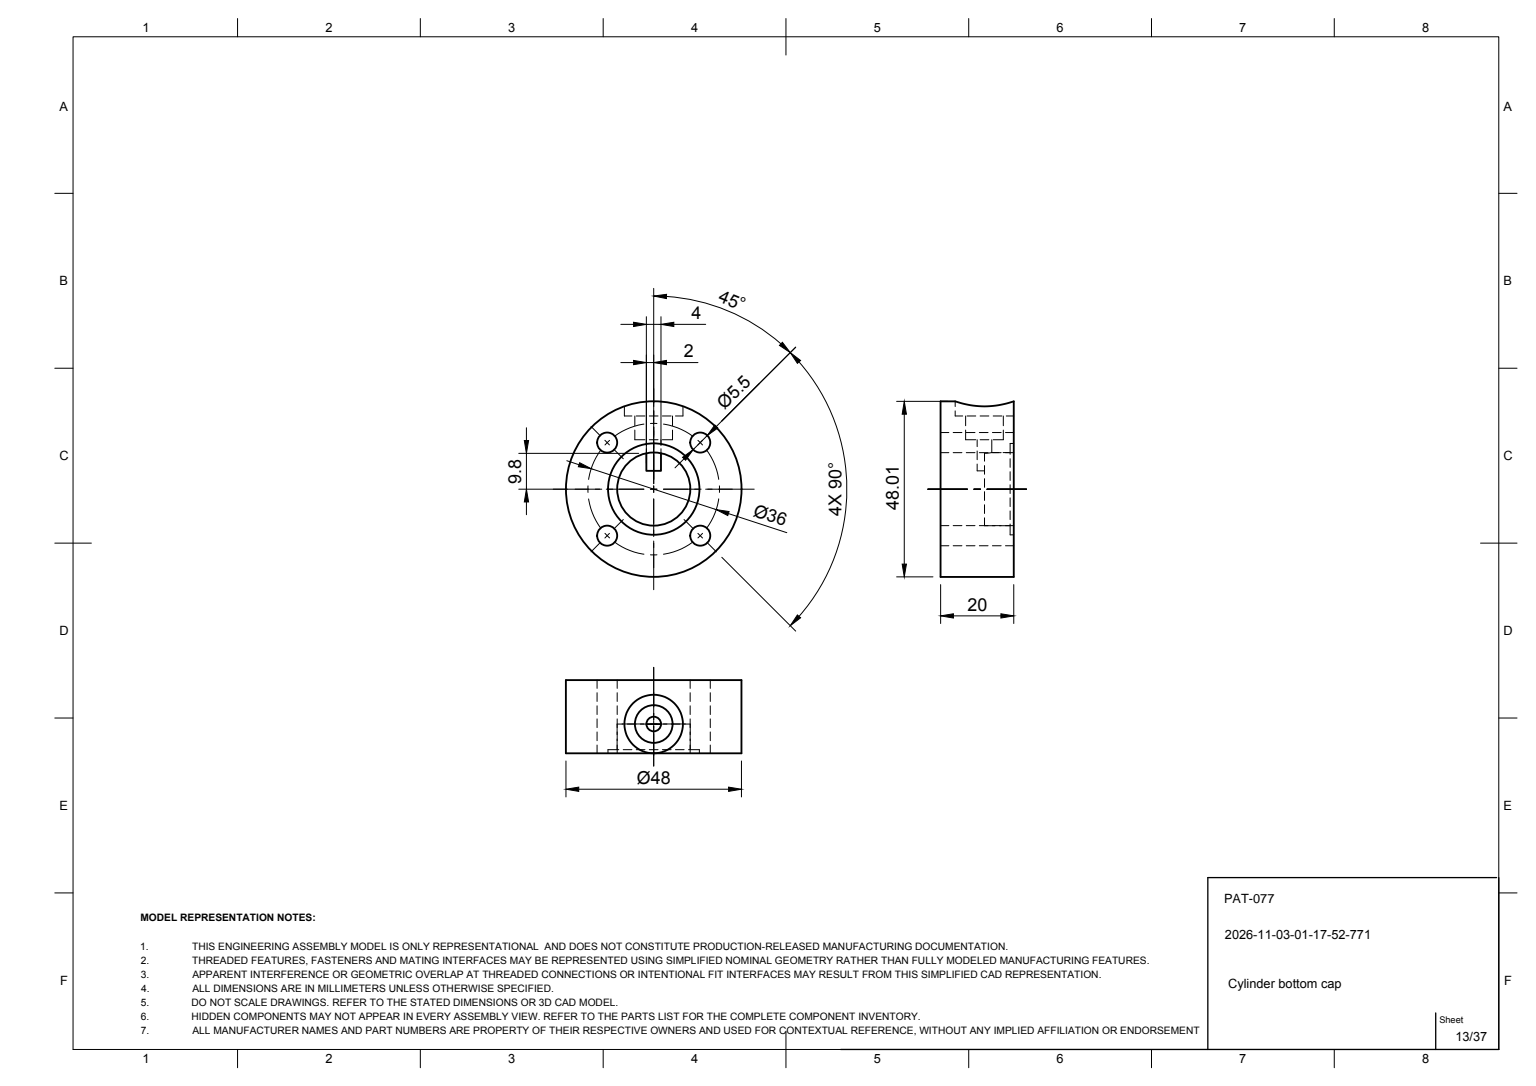
ISO-10303-21;
HEADER;
/* Generated by software containing ST-Developer
 * from STEP Tools, Inc. (www.steptools.com) 
 */

FILE_DESCRIPTION(
/* description */ ('Pallet stop with pneumatic fitting'),
/* implementation_level */ '2;1');

FILE_NAME(
/* name */ 'Cylinder bottom cap.step',
/* time_stamp */ '2026-10-27T10:51:41-07:00',
/* author */ (''),
/* organization */ (''),
/* preprocessor_version */ 'ST-DEVELOPER v20.2',
/* originating_system */ 'Autodesk Translation Framework v15.17.0.0',
/* authorisation */ '');

FILE_SCHEMA (('AUTOMOTIVE_DESIGN { 1 0 10303 214 3 1 1 }'));
ENDSEC;

DATA;
#10=MECHANICAL_DESIGN_GEOMETRIC_PRESENTATION_REPRESENTATION('',(#365),#10265);
#281=B_SPLINE_CURVE_WITH_KNOTS('',3,(#8964,#8965,#8966,#8967,#8968,#8969,
#8970,#8971,#8972,#8973,#8974,#8975,#8976,#8977,#8978,#8979,#8980,#8981,
#8982,#8983,#8984,#8985,#8986,#8987,#8988,#8989),.UNSPECIFIED.,.F.,.F.,
(4,2,2,2,2,2,2,2,2,2,2,2,4),(4.86208093968474,5.16603148466369,5.46998202964264,
5.77379160212428,6.07760117460592,6.38141074708757,6.68522031956921,6.98917086454816,
7.29312140952711,7.59707195450606,7.90102249948501,8.20483207196665,8.50864164444829),
 .UNSPECIFIED.);
#282=B_SPLINE_CURVE_WITH_KNOTS('',3,(#8999,#9000,#9001,#9002,#9003,#9004,
#9005,#9006,#9007,#9008,#9009,#9010,#9011,#9012,#9013,#9014,#9015,#9016),
 .UNSPECIFIED.,.F.,.F.,(4,2,2,2,2,2,2,2,4),(0.,0.0755590511780388,0.151118102356078,
0.226672919608918,0.302227736861757,0.377782554114597,0.453337371367437,
0.528896422545476,0.604455473723515),.UNSPECIFIED.);
#283=B_SPLINE_CURVE_WITH_KNOTS('',3,(#9033,#9034,#9035,#9036,#9037,#9038,
#9039,#9040,#9041,#9042),.UNSPECIFIED.,.F.,.F.,(4,2,2,2,4),(3.64656070476355,
3.9503702772452,4.25417984972684,4.55813039470579,4.86208093968474),
 .UNSPECIFIED.);
#301=SHAPE_REPRESENTATION_RELATIONSHIP('SRR','None',#10414,#333);
#333=ADVANCED_BREP_SHAPE_REPRESENTATION('',(#397),#10238);
#365=STYLED_ITEM('',(#10648),#397);
#397=MANIFOLD_SOLID_BREP('Body1',#5053);
#466=FACE_BOUND('',#1191,.T.);
#467=FACE_BOUND('',#1194,.T.);
#468=FACE_BOUND('',#1198,.T.);
#469=FACE_BOUND('',#1205,.T.);
#470=FACE_BOUND('',#1206,.T.);
#471=FACE_BOUND('',#1207,.T.);
#472=FACE_BOUND('',#1208,.T.);
#473=FACE_BOUND('',#1209,.T.);
#474=FACE_BOUND('',#1211,.T.);
#475=FACE_BOUND('',#1212,.T.);
#476=FACE_BOUND('',#1213,.T.);
#477=FACE_BOUND('',#1214,.T.);
#599=PLANE('',#5600);
#600=PLANE('',#5604);
#601=PLANE('',#5610);
#602=PLANE('',#5613);
#603=PLANE('',#5621);
#604=PLANE('',#5636);
#605=PLANE('',#5637);
#824=FACE_OUTER_BOUND('',#1185,.T.);
#825=FACE_OUTER_BOUND('',#1186,.T.);
#826=FACE_OUTER_BOUND('',#1187,.T.);
#827=FACE_OUTER_BOUND('',#1188,.T.);
#828=FACE_OUTER_BOUND('',#1189,.T.);
#829=FACE_OUTER_BOUND('',#1190,.T.);
#830=FACE_OUTER_BOUND('',#1192,.T.);
#831=FACE_OUTER_BOUND('',#1193,.T.);
#832=FACE_OUTER_BOUND('',#1195,.T.);
#833=FACE_OUTER_BOUND('',#1196,.T.);
#834=FACE_OUTER_BOUND('',#1197,.T.);
#835=FACE_OUTER_BOUND('',#1199,.T.);
#836=FACE_OUTER_BOUND('',#1200,.T.);
#837=FACE_OUTER_BOUND('',#1201,.T.);
#838=FACE_OUTER_BOUND('',#1202,.T.);
#839=FACE_OUTER_BOUND('',#1203,.T.);
#840=FACE_OUTER_BOUND('',#1204,.T.);
#841=FACE_OUTER_BOUND('',#1210,.T.);
#1185=EDGE_LOOP('',(#3752,#3753,#3754,#3755));
#1186=EDGE_LOOP('',(#3756,#3757));
#1187=EDGE_LOOP('',(#3758,#3759,#3760,#3761,#3762,#3763,#3764));
#1188=EDGE_LOOP('',(#3765,#3766,#3767,#3768,#3769));
#1189=EDGE_LOOP('',(#3770,#3771,#3772,#3773));
#1190=EDGE_LOOP('',(#3774));
#1191=EDGE_LOOP('',(#3775));
#1192=EDGE_LOOP('',(#3776,#3777,#3778,#3779));
#1193=EDGE_LOOP('',(#3780,#3781));
#1194=EDGE_LOOP('',(#3782));
#1195=EDGE_LOOP('',(#3783,#3784,#3785,#3786,#3787,#3788,#3789));
#1196=EDGE_LOOP('',(#3790,#3791,#3792,#3793));
#1197=EDGE_LOOP('',(#3794));
#1198=EDGE_LOOP('',(#3795));
#1199=EDGE_LOOP('',(#3796,#3797,#3798,#3799,#3800,#3801));
#1200=EDGE_LOOP('',(#3802,#3803,#3804,#3805));
#1201=EDGE_LOOP('',(#3806,#3807,#3808,#3809));
#1202=EDGE_LOOP('',(#3810,#3811,#3812,#3813));
#1203=EDGE_LOOP('',(#3814,#3815,#3816,#3817));
#1204=EDGE_LOOP('',(#3818,#3819,#3820,#3821));
#1205=EDGE_LOOP('',(#3822));
#1206=EDGE_LOOP('',(#3823));
#1207=EDGE_LOOP('',(#3824));
#1208=EDGE_LOOP('',(#3825));
#1209=EDGE_LOOP('',(#3826));
#1210=EDGE_LOOP('',(#3827));
#1211=EDGE_LOOP('',(#3828));
#1212=EDGE_LOOP('',(#3829));
#1213=EDGE_LOOP('',(#3830));
#1214=EDGE_LOOP('',(#3831));
#1592=LINE('',#8959,#1927);
#1593=LINE('',#8963,#1928);
#1594=LINE('',#8993,#1929);
#1595=LINE('',#8997,#1930);
#1596=LINE('',#9018,#1931);
#1597=LINE('',#9020,#1932);
#1598=LINE('',#9029,#1933);
#1599=LINE('',#9043,#1934);
#1600=LINE('',#9051,#1935);
#1601=LINE('',#9057,#1936);
#1602=LINE('',#9063,#1937);
#1603=LINE('',#9068,#1938);
#1604=LINE('',#9074,#1939);
#1605=LINE('',#9080,#1940);
#1606=LINE('',#9086,#1941);
#1927=VECTOR('',#6525,0.8);
#1928=VECTOR('',#6528,1.);
#1929=VECTOR('',#6531,1.);
#1930=VECTOR('',#6536,1.);
#1931=VECTOR('',#6537,0.2);
#1932=VECTOR('',#6540,1.);
#1933=VECTOR('',#6551,0.515);
#1934=VECTOR('',#6558,1.);
#1935=VECTOR('',#6569,2.4);
#1936=VECTOR('',#6576,1.25);
#1937=VECTOR('',#6585,1.);
#1938=VECTOR('',#6590,0.275);
#1939=VECTOR('',#6597,0.275);
#1940=VECTOR('',#6604,0.275);
#1941=VECTOR('',#6611,0.275);
#2228=CIRCLE('',#5599,0.8);
#2229=CIRCLE('',#5601,0.2);
#2230=CIRCLE('',#5603,0.2);
#2231=CIRCLE('',#5605,1.);
#2232=CIRCLE('',#5606,1.);
#2233=CIRCLE('',#5608,0.515);
#2234=CIRCLE('',#5609,0.515);
#2235=CIRCLE('',#5612,0.8);
#2236=CIRCLE('',#5615,2.4);
#2237=CIRCLE('',#5616,2.4);
#2238=CIRCLE('',#5617,2.4);
#2239=CIRCLE('',#5619,1.25);
#2240=CIRCLE('',#5620,1.25);
#2241=CIRCLE('',#5622,1.);
#2242=CIRCLE('',#5625,0.275);
#2243=CIRCLE('',#5626,0.275);
#2244=CIRCLE('',#5628,0.275);
#2245=CIRCLE('',#5629,0.275);
#2246=CIRCLE('',#5631,0.275);
#2247=CIRCLE('',#5632,0.275);
#2248=CIRCLE('',#5634,0.275);
#2249=CIRCLE('',#5635,0.275);
#2521=VERTEX_POINT('',#8957);
#2522=VERTEX_POINT('',#8958);
#2523=VERTEX_POINT('',#8960);
#2524=VERTEX_POINT('',#8962);
#2525=VERTEX_POINT('',#8991);
#2526=VERTEX_POINT('',#8992);
#2527=VERTEX_POINT('',#8996);
#2528=VERTEX_POINT('',#8998);
#2529=VERTEX_POINT('',#9017);
#2530=VERTEX_POINT('',#9022);
#2531=VERTEX_POINT('',#9026);
#2532=VERTEX_POINT('',#9028);
#2533=VERTEX_POINT('',#9047);
#2534=VERTEX_POINT('',#9050);
#2535=VERTEX_POINT('',#9054);
#2536=VERTEX_POINT('',#9056);
#2537=VERTEX_POINT('',#9060);
#2538=VERTEX_POINT('',#9065);
#2539=VERTEX_POINT('',#9067);
#2540=VERTEX_POINT('',#9071);
#2541=VERTEX_POINT('',#9073);
#2542=VERTEX_POINT('',#9077);
#2543=VERTEX_POINT('',#9079);
#2544=VERTEX_POINT('',#9083);
#2545=VERTEX_POINT('',#9085);
#2975=EDGE_CURVE('',#2521,#2522,#1592,.T.);
#2976=EDGE_CURVE('',#2523,#2521,#2228,.T.);
#2977=EDGE_CURVE('',#2523,#2524,#1593,.T.);
#2978=EDGE_CURVE('',#2522,#2524,#281,.T.);
#2979=EDGE_CURVE('',#2525,#2526,#1594,.T.);
#2980=EDGE_CURVE('',#2525,#2526,#2229,.T.);
#2981=EDGE_CURVE('',#2527,#2525,#1595,.T.);
#2982=EDGE_CURVE('',#2528,#2527,#282,.T.);
#2983=EDGE_CURVE('',#2528,#2529,#1596,.T.);
#2984=EDGE_CURVE('',#2529,#2529,#2230,.T.);
#2985=EDGE_CURVE('',#2526,#2528,#1597,.T.);
#2986=EDGE_CURVE('',#2528,#2530,#2231,.T.);
#2987=EDGE_CURVE('',#2530,#2527,#2232,.T.);
#2988=EDGE_CURVE('',#2531,#2531,#2233,.T.);
#2989=EDGE_CURVE('',#2531,#2532,#1598,.T.);
#2990=EDGE_CURVE('',#2532,#2532,#2234,.T.);
#2991=EDGE_CURVE('',#2524,#2522,#283,.T.);
#2992=EDGE_CURVE('',#2523,#2524,#1599,.T.);
#2993=EDGE_CURVE('',#2521,#2523,#2235,.T.);
#2994=EDGE_CURVE('',#2524,#2533,#2236,.T.);
#2995=EDGE_CURVE('',#2533,#2524,#2237,.T.);
#2996=EDGE_CURVE('',#2533,#2534,#1600,.T.);
#2997=EDGE_CURVE('',#2534,#2534,#2238,.T.);
#2998=EDGE_CURVE('',#2535,#2535,#2239,.T.);
#2999=EDGE_CURVE('',#2535,#2536,#1601,.T.);
#3000=EDGE_CURVE('',#2536,#2536,#2240,.T.);
#3001=EDGE_CURVE('',#2537,#2537,#2241,.T.);
#3002=EDGE_CURVE('',#2530,#2537,#1602,.T.);
#3003=EDGE_CURVE('',#2538,#2538,#2242,.T.);
#3004=EDGE_CURVE('',#2538,#2539,#1603,.T.);
#3005=EDGE_CURVE('',#2539,#2539,#2243,.T.);
#3006=EDGE_CURVE('',#2540,#2540,#2244,.T.);
#3007=EDGE_CURVE('',#2540,#2541,#1604,.T.);
#3008=EDGE_CURVE('',#2541,#2541,#2245,.T.);
#3009=EDGE_CURVE('',#2542,#2542,#2246,.T.);
#3010=EDGE_CURVE('',#2542,#2543,#1605,.T.);
#3011=EDGE_CURVE('',#2543,#2543,#2247,.T.);
#3012=EDGE_CURVE('',#2544,#2544,#2248,.T.);
#3013=EDGE_CURVE('',#2544,#2545,#1606,.T.);
#3014=EDGE_CURVE('',#2545,#2545,#2249,.T.);
#3752=ORIENTED_EDGE('',*,*,#2975,.F.);
#3753=ORIENTED_EDGE('',*,*,#2976,.F.);
#3754=ORIENTED_EDGE('',*,*,#2977,.T.);
#3755=ORIENTED_EDGE('',*,*,#2978,.F.);
#3756=ORIENTED_EDGE('',*,*,#2979,.F.);
#3757=ORIENTED_EDGE('',*,*,#2980,.T.);
#3758=ORIENTED_EDGE('',*,*,#2981,.F.);
#3759=ORIENTED_EDGE('',*,*,#2982,.F.);
#3760=ORIENTED_EDGE('',*,*,#2983,.T.);
#3761=ORIENTED_EDGE('',*,*,#2984,.F.);
#3762=ORIENTED_EDGE('',*,*,#2983,.F.);
#3763=ORIENTED_EDGE('',*,*,#2985,.F.);
#3764=ORIENTED_EDGE('',*,*,#2980,.F.);
#3765=ORIENTED_EDGE('',*,*,#2981,.T.);
#3766=ORIENTED_EDGE('',*,*,#2979,.T.);
#3767=ORIENTED_EDGE('',*,*,#2985,.T.);
#3768=ORIENTED_EDGE('',*,*,#2986,.T.);
#3769=ORIENTED_EDGE('',*,*,#2987,.T.);
#3770=ORIENTED_EDGE('',*,*,#2988,.F.);
#3771=ORIENTED_EDGE('',*,*,#2989,.T.);
#3772=ORIENTED_EDGE('',*,*,#2990,.F.);
#3773=ORIENTED_EDGE('',*,*,#2989,.F.);
#3774=ORIENTED_EDGE('',*,*,#2988,.T.);
#3775=ORIENTED_EDGE('',*,*,#2984,.T.);
#3776=ORIENTED_EDGE('',*,*,#2975,.T.);
#3777=ORIENTED_EDGE('',*,*,#2991,.F.);
#3778=ORIENTED_EDGE('',*,*,#2992,.F.);
#3779=ORIENTED_EDGE('',*,*,#2993,.F.);
#3780=ORIENTED_EDGE('',*,*,#2976,.T.);
#3781=ORIENTED_EDGE('',*,*,#2993,.T.);
#3782=ORIENTED_EDGE('',*,*,#2990,.T.);
#3783=ORIENTED_EDGE('',*,*,#2994,.F.);
#3784=ORIENTED_EDGE('',*,*,#2991,.T.);
#3785=ORIENTED_EDGE('',*,*,#2978,.T.);
#3786=ORIENTED_EDGE('',*,*,#2995,.F.);
#3787=ORIENTED_EDGE('',*,*,#2996,.T.);
#3788=ORIENTED_EDGE('',*,*,#2997,.T.);
#3789=ORIENTED_EDGE('',*,*,#2996,.F.);
#3790=ORIENTED_EDGE('',*,*,#2998,.F.);
#3791=ORIENTED_EDGE('',*,*,#2999,.T.);
#3792=ORIENTED_EDGE('',*,*,#3000,.F.);
#3793=ORIENTED_EDGE('',*,*,#2999,.F.);
#3794=ORIENTED_EDGE('',*,*,#2998,.T.);
#3795=ORIENTED_EDGE('',*,*,#3001,.F.);
#3796=ORIENTED_EDGE('',*,*,#2982,.T.);
#3797=ORIENTED_EDGE('',*,*,#2987,.F.);
#3798=ORIENTED_EDGE('',*,*,#3002,.T.);
#3799=ORIENTED_EDGE('',*,*,#3001,.T.);
#3800=ORIENTED_EDGE('',*,*,#3002,.F.);
#3801=ORIENTED_EDGE('',*,*,#2986,.F.);
#3802=ORIENTED_EDGE('',*,*,#3003,.F.);
#3803=ORIENTED_EDGE('',*,*,#3004,.T.);
#3804=ORIENTED_EDGE('',*,*,#3005,.F.);
#3805=ORIENTED_EDGE('',*,*,#3004,.F.);
#3806=ORIENTED_EDGE('',*,*,#3006,.F.);
#3807=ORIENTED_EDGE('',*,*,#3007,.T.);
#3808=ORIENTED_EDGE('',*,*,#3008,.F.);
#3809=ORIENTED_EDGE('',*,*,#3007,.F.);
#3810=ORIENTED_EDGE('',*,*,#3009,.F.);
#3811=ORIENTED_EDGE('',*,*,#3010,.T.);
#3812=ORIENTED_EDGE('',*,*,#3011,.F.);
#3813=ORIENTED_EDGE('',*,*,#3010,.F.);
#3814=ORIENTED_EDGE('',*,*,#3012,.F.);
#3815=ORIENTED_EDGE('',*,*,#3013,.T.);
#3816=ORIENTED_EDGE('',*,*,#3014,.F.);
#3817=ORIENTED_EDGE('',*,*,#3013,.F.);
#3818=ORIENTED_EDGE('',*,*,#2994,.T.);
#3819=ORIENTED_EDGE('',*,*,#2995,.T.);
#3820=ORIENTED_EDGE('',*,*,#2977,.F.);
#3821=ORIENTED_EDGE('',*,*,#2992,.T.);
#3822=ORIENTED_EDGE('',*,*,#3000,.T.);
#3823=ORIENTED_EDGE('',*,*,#3005,.T.);
#3824=ORIENTED_EDGE('',*,*,#3008,.T.);
#3825=ORIENTED_EDGE('',*,*,#3011,.T.);
#3826=ORIENTED_EDGE('',*,*,#3014,.T.);
#3827=ORIENTED_EDGE('',*,*,#2997,.F.);
#3828=ORIENTED_EDGE('',*,*,#3003,.T.);
#3829=ORIENTED_EDGE('',*,*,#3006,.T.);
#3830=ORIENTED_EDGE('',*,*,#3009,.T.);
#3831=ORIENTED_EDGE('',*,*,#3012,.T.);
#4655=CYLINDRICAL_SURFACE('',#5598,0.8);
#4656=CYLINDRICAL_SURFACE('',#5602,0.2);
#4657=CYLINDRICAL_SURFACE('',#5607,0.515);
#4658=CYLINDRICAL_SURFACE('',#5611,0.8);
#4659=CYLINDRICAL_SURFACE('',#5614,2.4);
#4660=CYLINDRICAL_SURFACE('',#5618,1.25);
#4661=CYLINDRICAL_SURFACE('',#5623,1.);
#4662=CYLINDRICAL_SURFACE('',#5624,0.275);
#4663=CYLINDRICAL_SURFACE('',#5627,0.275);
#4664=CYLINDRICAL_SURFACE('',#5630,0.275);
#4665=CYLINDRICAL_SURFACE('',#5633,0.275);
#4819=ADVANCED_FACE('',(#824),#4655,.F.);
#4820=ADVANCED_FACE('',(#825),#599,.T.);
#4821=ADVANCED_FACE('',(#826),#4656,.F.);
#4822=ADVANCED_FACE('',(#827),#600,.T.);
#4823=ADVANCED_FACE('',(#828),#4657,.F.);
#4824=ADVANCED_FACE('',(#829,#466),#601,.T.);
#4825=ADVANCED_FACE('',(#830),#4658,.F.);
#4826=ADVANCED_FACE('',(#831,#467),#602,.T.);
#4827=ADVANCED_FACE('',(#832),#4659,.T.);
#4828=ADVANCED_FACE('',(#833),#4660,.F.);
#4829=ADVANCED_FACE('',(#834,#468),#603,.T.);
#4830=ADVANCED_FACE('',(#835),#4661,.F.);
#4831=ADVANCED_FACE('',(#836),#4662,.F.);
#4832=ADVANCED_FACE('',(#837),#4663,.F.);
#4833=ADVANCED_FACE('',(#838),#4664,.F.);
#4834=ADVANCED_FACE('',(#839),#4665,.F.);
#4835=ADVANCED_FACE('',(#840,#469,#470,#471,#472,#473),#604,.T.);
#4836=ADVANCED_FACE('',(#841,#474,#475,#476,#477),#605,.F.);
#5053=CLOSED_SHELL('',(#4819,#4820,#4821,#4822,#4823,#4824,#4825,#4826,
#4827,#4828,#4829,#4830,#4831,#4832,#4833,#4834,#4835,#4836));
#5597=AXIS2_PLACEMENT_3D('',#8955,#6521,#6522);
#5598=AXIS2_PLACEMENT_3D('',#8956,#6523,#6524);
#5599=AXIS2_PLACEMENT_3D('',#8961,#6526,#6527);
#5600=AXIS2_PLACEMENT_3D('',#8990,#6529,#6530);
#5601=AXIS2_PLACEMENT_3D('',#8994,#6532,#6533);
#5602=AXIS2_PLACEMENT_3D('',#8995,#6534,#6535);
#5603=AXIS2_PLACEMENT_3D('',#9019,#6538,#6539);
#5604=AXIS2_PLACEMENT_3D('',#9021,#6541,#6542);
#5605=AXIS2_PLACEMENT_3D('',#9023,#6543,#6544);
#5606=AXIS2_PLACEMENT_3D('',#9024,#6545,#6546);
#5607=AXIS2_PLACEMENT_3D('',#9025,#6547,#6548);
#5608=AXIS2_PLACEMENT_3D('',#9027,#6549,#6550);
#5609=AXIS2_PLACEMENT_3D('',#9030,#6552,#6553);
#5610=AXIS2_PLACEMENT_3D('',#9031,#6554,#6555);
#5611=AXIS2_PLACEMENT_3D('',#9032,#6556,#6557);
#5612=AXIS2_PLACEMENT_3D('',#9044,#6559,#6560);
#5613=AXIS2_PLACEMENT_3D('',#9045,#6561,#6562);
#5614=AXIS2_PLACEMENT_3D('',#9046,#6563,#6564);
#5615=AXIS2_PLACEMENT_3D('',#9048,#6565,#6566);
#5616=AXIS2_PLACEMENT_3D('',#9049,#6567,#6568);
#5617=AXIS2_PLACEMENT_3D('',#9052,#6570,#6571);
#5618=AXIS2_PLACEMENT_3D('',#9053,#6572,#6573);
#5619=AXIS2_PLACEMENT_3D('',#9055,#6574,#6575);
#5620=AXIS2_PLACEMENT_3D('',#9058,#6577,#6578);
#5621=AXIS2_PLACEMENT_3D('',#9059,#6579,#6580);
#5622=AXIS2_PLACEMENT_3D('',#9061,#6581,#6582);
#5623=AXIS2_PLACEMENT_3D('',#9062,#6583,#6584);
#5624=AXIS2_PLACEMENT_3D('',#9064,#6586,#6587);
#5625=AXIS2_PLACEMENT_3D('',#9066,#6588,#6589);
#5626=AXIS2_PLACEMENT_3D('',#9069,#6591,#6592);
#5627=AXIS2_PLACEMENT_3D('',#9070,#6593,#6594);
#5628=AXIS2_PLACEMENT_3D('',#9072,#6595,#6596);
#5629=AXIS2_PLACEMENT_3D('',#9075,#6598,#6599);
#5630=AXIS2_PLACEMENT_3D('',#9076,#6600,#6601);
#5631=AXIS2_PLACEMENT_3D('',#9078,#6602,#6603);
#5632=AXIS2_PLACEMENT_3D('',#9081,#6605,#6606);
#5633=AXIS2_PLACEMENT_3D('',#9082,#6607,#6608);
#5634=AXIS2_PLACEMENT_3D('',#9084,#6609,#6610);
#5635=AXIS2_PLACEMENT_3D('',#9087,#6612,#6613);
#5636=AXIS2_PLACEMENT_3D('',#9088,#6614,#6615);
#5637=AXIS2_PLACEMENT_3D('',#9089,#6616,#6617);
#6521=DIRECTION('axis',(0.,0.,1.));
#6522=DIRECTION('refdir',(1.,0.,0.));
#6523=DIRECTION('center_axis',(0.,1.,0.));
#6524=DIRECTION('ref_axis',(1.,0.,0.));
#6525=DIRECTION('',(0.,1.,0.));
#6526=DIRECTION('center_axis',(0.,1.,0.));
#6527=DIRECTION('ref_axis',(1.,0.,0.));
#6528=DIRECTION('',(0.,1.,0.));
#6529=DIRECTION('center_axis',(0.,1.,0.));
#6530=DIRECTION('ref_axis',(1.,0.,0.));
#6531=DIRECTION('',(-1.,0.,0.));
#6532=DIRECTION('center_axis',(0.,1.,0.));
#6533=DIRECTION('ref_axis',(1.,0.,0.));
#6534=DIRECTION('center_axis',(0.,1.,0.));
#6535=DIRECTION('ref_axis',(1.,0.,0.));
#6536=DIRECTION('',(0.,-1.,0.));
#6537=DIRECTION('',(0.,1.,0.));
#6538=DIRECTION('center_axis',(0.,-1.,0.));
#6539=DIRECTION('ref_axis',(1.,0.,0.));
#6540=DIRECTION('',(0.,1.,0.));
#6541=DIRECTION('center_axis',(0.,0.,1.));
#6542=DIRECTION('ref_axis',(1.,0.,0.));
#6543=DIRECTION('center_axis',(0.,0.,1.));
#6544=DIRECTION('ref_axis',(1.,0.,0.));
#6545=DIRECTION('center_axis',(0.,0.,1.));
#6546=DIRECTION('ref_axis',(1.,0.,0.));
#6547=DIRECTION('center_axis',(0.,1.,0.));
#6548=DIRECTION('ref_axis',(1.,0.,0.));
#6549=DIRECTION('center_axis',(0.,1.,0.));
#6550=DIRECTION('ref_axis',(1.,0.,0.));
#6551=DIRECTION('',(0.,1.,0.));
#6552=DIRECTION('center_axis',(0.,-1.,0.));
#6553=DIRECTION('ref_axis',(1.,0.,0.));
#6554=DIRECTION('center_axis',(0.,1.,0.));
#6555=DIRECTION('ref_axis',(1.,0.,0.));
#6556=DIRECTION('center_axis',(0.,1.,0.));
#6557=DIRECTION('ref_axis',(1.,0.,0.));
#6558=DIRECTION('',(0.,1.,0.));
#6559=DIRECTION('center_axis',(0.,1.,0.));
#6560=DIRECTION('ref_axis',(1.,0.,0.));
#6561=DIRECTION('center_axis',(0.,1.,0.));
#6562=DIRECTION('ref_axis',(1.,0.,0.));
#6563=DIRECTION('center_axis',(0.,0.,1.));
#6564=DIRECTION('ref_axis',(1.,0.,0.));
#6565=DIRECTION('center_axis',(0.,0.,1.));
#6566=DIRECTION('ref_axis',(1.,0.,0.));
#6567=DIRECTION('center_axis',(0.,0.,1.));
#6568=DIRECTION('ref_axis',(1.,0.,0.));
#6569=DIRECTION('',(0.,0.,-1.));
#6570=DIRECTION('center_axis',(0.,0.,1.));
#6571=DIRECTION('ref_axis',(1.,0.,0.));
#6572=DIRECTION('center_axis',(0.,0.,1.));
#6573=DIRECTION('ref_axis',(1.,0.,0.));
#6574=DIRECTION('center_axis',(0.,0.,1.));
#6575=DIRECTION('ref_axis',(1.,0.,0.));
#6576=DIRECTION('',(0.,0.,1.));
#6577=DIRECTION('center_axis',(0.,0.,-1.));
#6578=DIRECTION('ref_axis',(1.,0.,0.));
#6579=DIRECTION('center_axis',(0.,0.,1.));
#6580=DIRECTION('ref_axis',(1.,0.,0.));
#6581=DIRECTION('center_axis',(0.,0.,1.));
#6582=DIRECTION('ref_axis',(1.,0.,0.));
#6583=DIRECTION('center_axis',(0.,0.,1.));
#6584=DIRECTION('ref_axis',(1.,0.,0.));
#6585=DIRECTION('',(0.,0.,1.));
#6586=DIRECTION('center_axis',(0.,0.,1.));
#6587=DIRECTION('ref_axis',(1.,0.,0.));
#6588=DIRECTION('center_axis',(0.,0.,1.));
#6589=DIRECTION('ref_axis',(1.,0.,0.));
#6590=DIRECTION('',(0.,0.,1.));
#6591=DIRECTION('center_axis',(0.,0.,-1.));
#6592=DIRECTION('ref_axis',(1.,0.,0.));
#6593=DIRECTION('center_axis',(0.,0.,1.));
#6594=DIRECTION('ref_axis',(1.,0.,0.));
#6595=DIRECTION('center_axis',(0.,0.,1.));
#6596=DIRECTION('ref_axis',(1.,0.,0.));
#6597=DIRECTION('',(0.,0.,1.));
#6598=DIRECTION('center_axis',(0.,0.,-1.));
#6599=DIRECTION('ref_axis',(1.,0.,0.));
#6600=DIRECTION('center_axis',(0.,0.,1.));
#6601=DIRECTION('ref_axis',(1.,0.,0.));
#6602=DIRECTION('center_axis',(0.,0.,1.));
#6603=DIRECTION('ref_axis',(1.,0.,0.));
#6604=DIRECTION('',(0.,0.,1.));
#6605=DIRECTION('center_axis',(0.,0.,-1.));
#6606=DIRECTION('ref_axis',(1.,0.,0.));
#6607=DIRECTION('center_axis',(0.,0.,1.));
#6608=DIRECTION('ref_axis',(1.,0.,0.));
#6609=DIRECTION('center_axis',(0.,0.,1.));
#6610=DIRECTION('ref_axis',(1.,0.,0.));
#6611=DIRECTION('',(0.,0.,1.));
#6612=DIRECTION('center_axis',(0.,0.,-1.));
#6613=DIRECTION('ref_axis',(1.,0.,0.));
#6614=DIRECTION('center_axis',(0.,0.,1.));
#6615=DIRECTION('ref_axis',(1.,0.,0.));
#6616=DIRECTION('center_axis',(0.,0.,1.));
#6617=DIRECTION('ref_axis',(1.,0.,0.));
#8955=CARTESIAN_POINT('',(0.,0.,0.));
#8956=CARTESIAN_POINT('Origin',(4.,6.,1.2));
#8957=CARTESIAN_POINT('',(3.2,6.,1.2));
#8958=CARTESIAN_POINT('',(3.2,6.26274169979695,1.2));
#8959=CARTESIAN_POINT('',(3.2,6.,1.2));
#8960=CARTESIAN_POINT('',(4.,6.,2.));
#8961=CARTESIAN_POINT('Origin',(4.,6.,1.2));
#8962=CARTESIAN_POINT('',(4.,6.4,2.));
#8963=CARTESIAN_POINT('',(4.,6.,2.));
#8964=CARTESIAN_POINT('Ctrl Pts',(3.2,6.26274169979695,1.2));
#8965=CARTESIAN_POINT('Ctrl Pts',(3.2,6.26274169979695,1.09868315167368));
#8966=CARTESIAN_POINT('Ctrl Pts',(3.22040772858495,6.270261426297,0.991198421229182));
#8967=CARTESIAN_POINT('Ctrl Pts',(3.30227767389892,6.29674433020986,0.794357456033841));
#8968=CARTESIAN_POINT('Ctrl Pts',(3.36370361600024,6.31525508485039,0.704925534101287));
#8969=CARTESIAN_POINT('Ctrl Pts',(3.50489278468399,6.34949848812546,0.563736365417532));
#8970=CARTESIAN_POINT('Ctrl Pts',(3.59433775043408,6.36754956424272,0.502285211106731));
#8971=CARTESIAN_POINT('Ctrl Pts',(3.79122709022331,6.39296190354765,0.420396463357562));
#8972=CARTESIAN_POINT('Ctrl Pts',(3.89873014250612,6.4,0.4));
#8973=CARTESIAN_POINT('Ctrl Pts',(4.10126985749388,6.4,0.4));
#8974=CARTESIAN_POINT('Ctrl Pts',(4.20877290977669,6.39296190354765,0.420396463357562));
#8975=CARTESIAN_POINT('Ctrl Pts',(4.40566224956592,6.36754956424272,0.502285211106731));
#8976=CARTESIAN_POINT('Ctrl Pts',(4.49510721531601,6.34949848812546,0.563736365417532));
#8977=CARTESIAN_POINT('Ctrl Pts',(4.63629638399976,6.31525508485039,0.704925534101287));
#8978=CARTESIAN_POINT('Ctrl Pts',(4.69772232610108,6.29674433020986,0.794357456033842));
#8979=CARTESIAN_POINT('Ctrl Pts',(4.77959227141505,6.270261426297,0.991198421229182));
#8980=CARTESIAN_POINT('Ctrl Pts',(4.8,6.26274169979695,1.09868315167368));
#8981=CARTESIAN_POINT('Ctrl Pts',(4.8,6.26274169979695,1.30131684832632));
#8982=CARTESIAN_POINT('Ctrl Pts',(4.77959227141505,6.270261426297,1.40880157877082));
#8983=CARTESIAN_POINT('Ctrl Pts',(4.69772232610108,6.29674433020986,1.60564254396616));
#8984=CARTESIAN_POINT('Ctrl Pts',(4.63629638399976,6.31525508485039,1.69507446589871));
#8985=CARTESIAN_POINT('Ctrl Pts',(4.49510721531601,6.34949848812546,1.83626363458247));
#8986=CARTESIAN_POINT('Ctrl Pts',(4.40566224956592,6.36754956424272,1.89771478889327));
#8987=CARTESIAN_POINT('Ctrl Pts',(4.20877290977668,6.39296190354765,1.97960353664244));
#8988=CARTESIAN_POINT('Ctrl Pts',(4.10126985749388,6.4,2.));
#8989=CARTESIAN_POINT('Ctrl Pts',(4.,6.4,2.));
#8990=CARTESIAN_POINT('Origin',(4.,4.5,1.2));
#8991=CARTESIAN_POINT('',(4.2,4.5,1.2));
#8992=CARTESIAN_POINT('',(3.8,4.5,1.2));
#8993=CARTESIAN_POINT('',(4.,4.5,1.2));
#8994=CARTESIAN_POINT('Origin',(4.,4.5,1.2));
#8995=CARTESIAN_POINT('Origin',(4.,4.5,1.2));
#8996=CARTESIAN_POINT('',(4.2,4.97979589711327,1.2));
#8997=CARTESIAN_POINT('',(4.2,4.5,1.2));
#8998=CARTESIAN_POINT('',(3.8,4.97979589711327,1.2));
#8999=CARTESIAN_POINT('Ctrl Pts',(3.8,4.97979589711327,1.2));
#9000=CARTESIAN_POINT('Ctrl Pts',(3.8,4.97979589711327,1.22518635039268));
#9001=CARTESIAN_POINT('Ctrl Pts',(3.80504744075028,4.98086775323689,1.25200355543238));
#9002=CARTESIAN_POINT('Ctrl Pts',(3.82547891647032,4.98470830158554,1.30125840100601));
#9003=CARTESIAN_POINT('Ctrl Pts',(3.84085937956158,4.98741817020387,1.3237020920362));
#9004=CARTESIAN_POINT('Ctrl Pts',(3.87629691507098,4.99248067527664,1.3591396275456));
#9005=CARTESIAN_POINT('Ctrl Pts',(3.89874102776047,4.99516669430373,1.37452086830895));
#9006=CARTESIAN_POINT('Ctrl Pts',(3.94799733878363,4.99895237729416,1.39495290844717));
#9007=CARTESIAN_POINT('Ctrl Pts',(3.97481506091572,5.,1.4));
#9008=CARTESIAN_POINT('Ctrl Pts',(4.02518493908428,5.,1.4));
#9009=CARTESIAN_POINT('Ctrl Pts',(4.05200266121637,4.99895237729416,1.39495290844717));
#9010=CARTESIAN_POINT('Ctrl Pts',(4.10125897223952,4.99516669430373,1.37452086830895));
#9011=CARTESIAN_POINT('Ctrl Pts',(4.12370308492902,4.99248067527664,1.3591396275456));
#9012=CARTESIAN_POINT('Ctrl Pts',(4.15914062043842,4.98741817020387,1.3237020920362));
#9013=CARTESIAN_POINT('Ctrl Pts',(4.17452108352968,4.98470830158554,1.30125840100601));
#9014=CARTESIAN_POINT('Ctrl Pts',(4.19495255924972,4.98086775323689,1.25200355543238));
#9015=CARTESIAN_POINT('Ctrl Pts',(4.2,4.97979589711327,1.22518635039268));
#9016=CARTESIAN_POINT('Ctrl Pts',(4.2,4.97979589711327,1.2));
#9017=CARTESIAN_POINT('',(3.8,5.35,1.2));
#9018=CARTESIAN_POINT('',(3.8,4.5,1.2));
#9019=CARTESIAN_POINT('Origin',(4.,5.35,1.2));
#9020=CARTESIAN_POINT('',(3.8,4.5,1.2));
#9021=CARTESIAN_POINT('Origin',(4.,4.,1.2));
#9022=CARTESIAN_POINT('',(3.,4.,1.2));
#9023=CARTESIAN_POINT('Origin',(4.,4.,1.2));
#9024=CARTESIAN_POINT('Origin',(4.,4.,1.2));
#9025=CARTESIAN_POINT('Origin',(4.,5.35,1.2));
#9026=CARTESIAN_POINT('',(3.485,5.35,1.2));
#9027=CARTESIAN_POINT('Origin',(4.,5.35,1.2));
#9028=CARTESIAN_POINT('',(3.485,6.,1.2));
#9029=CARTESIAN_POINT('',(3.485,5.35,1.2));
#9030=CARTESIAN_POINT('Origin',(4.,6.,1.2));
#9031=CARTESIAN_POINT('Origin',(4.,5.35,1.2));
#9032=CARTESIAN_POINT('Origin',(4.,6.,1.2));
#9033=CARTESIAN_POINT('Ctrl Pts',(4.,6.4,2.));
#9034=CARTESIAN_POINT('Ctrl Pts',(3.89873014250612,6.4,2.));
#9035=CARTESIAN_POINT('Ctrl Pts',(3.79122709022331,6.39296190354765,1.97960353664244));
#9036=CARTESIAN_POINT('Ctrl Pts',(3.59433775043408,6.36754956424272,1.89771478889327));
#9037=CARTESIAN_POINT('Ctrl Pts',(3.50489278468399,6.34949848812546,1.83626363458247));
#9038=CARTESIAN_POINT('Ctrl Pts',(3.36370361600024,6.31525508485039,1.69507446589871));
#9039=CARTESIAN_POINT('Ctrl Pts',(3.30227767389892,6.29674433020986,1.60564254396616));
#9040=CARTESIAN_POINT('Ctrl Pts',(3.22040772858495,6.270261426297,1.40880157877082));
#9041=CARTESIAN_POINT('Ctrl Pts',(3.2,6.26274169979695,1.30131684832632));
#9042=CARTESIAN_POINT('Ctrl Pts',(3.2,6.26274169979695,1.2));
#9043=CARTESIAN_POINT('',(4.,6.,2.));
#9044=CARTESIAN_POINT('Origin',(4.,6.,1.2));
#9045=CARTESIAN_POINT('Origin',(4.,6.,1.2));
#9046=CARTESIAN_POINT('Origin',(4.,4.,0.));
#9047=CARTESIAN_POINT('',(1.6,4.,2.));
#9048=CARTESIAN_POINT('Origin',(4.,4.,2.));
#9049=CARTESIAN_POINT('Origin',(4.,4.,2.));
#9050=CARTESIAN_POINT('',(1.6,4.,0.));
#9051=CARTESIAN_POINT('',(1.6,4.,0.));
#9052=CARTESIAN_POINT('Origin',(4.,4.,0.));
#9053=CARTESIAN_POINT('Origin',(4.,4.,1.9));
#9054=CARTESIAN_POINT('',(2.75,4.,1.9));
#9055=CARTESIAN_POINT('Origin',(4.,4.,1.9));
#9056=CARTESIAN_POINT('',(2.75,4.,2.));
#9057=CARTESIAN_POINT('',(2.75,4.,1.9));
#9058=CARTESIAN_POINT('Origin',(4.,4.,2.));
#9059=CARTESIAN_POINT('Origin',(4.,4.,1.9));
#9060=CARTESIAN_POINT('',(3.,4.,1.9));
#9061=CARTESIAN_POINT('Origin',(4.,4.,1.9));
#9062=CARTESIAN_POINT('Origin',(4.,4.,1.2));
#9063=CARTESIAN_POINT('',(3.,4.,1.2));
#9064=CARTESIAN_POINT('Origin',(2.72720779386421,2.72720779386421,-0.1));
#9065=CARTESIAN_POINT('',(2.45220779386421,2.72720779386421,0.));
#9066=CARTESIAN_POINT('Origin',(2.72720779386421,2.72720779386421,0.));
#9067=CARTESIAN_POINT('',(2.45220779386421,2.72720779386421,2.));
#9068=CARTESIAN_POINT('',(2.45220779386421,2.72720779386421,-0.1));
#9069=CARTESIAN_POINT('Origin',(2.72720779386421,2.72720779386421,2.));
#9070=CARTESIAN_POINT('Origin',(2.72720779386421,5.27279220613579,-0.1));
#9071=CARTESIAN_POINT('',(2.45220779386421,5.27279220613579,0.));
#9072=CARTESIAN_POINT('Origin',(2.72720779386421,5.27279220613579,0.));
#9073=CARTESIAN_POINT('',(2.45220779386421,5.27279220613579,2.));
#9074=CARTESIAN_POINT('',(2.45220779386421,5.27279220613579,-0.1));
#9075=CARTESIAN_POINT('Origin',(2.72720779386421,5.27279220613579,2.));
#9076=CARTESIAN_POINT('Origin',(5.27279220613579,5.27279220613579,-0.1));
#9077=CARTESIAN_POINT('',(4.99779220613579,5.27279220613579,0.));
#9078=CARTESIAN_POINT('Origin',(5.27279220613579,5.27279220613579,0.));
#9079=CARTESIAN_POINT('',(4.99779220613579,5.27279220613579,2.));
#9080=CARTESIAN_POINT('',(4.99779220613579,5.27279220613579,-0.1));
#9081=CARTESIAN_POINT('Origin',(5.27279220613579,5.27279220613579,2.));
#9082=CARTESIAN_POINT('Origin',(5.27279220613578,2.72720779386421,-0.1));
#9083=CARTESIAN_POINT('',(4.99779220613578,2.72720779386421,0.));
#9084=CARTESIAN_POINT('Origin',(5.27279220613578,2.72720779386421,0.));
#9085=CARTESIAN_POINT('',(4.99779220613578,2.72720779386421,2.));
#9086=CARTESIAN_POINT('',(4.99779220613578,2.72720779386421,-0.1));
#9087=CARTESIAN_POINT('Origin',(5.27279220613578,2.72720779386421,2.));
#9088=CARTESIAN_POINT('Origin',(4.,4.,2.));
#9089=CARTESIAN_POINT('Origin',(4.,4.,0.));
#10200=UNCERTAINTY_MEASURE_WITH_UNIT(LENGTH_MEASURE(0.001),#10266,
'DISTANCE_ACCURACY_VALUE',
'Maximum model space distance between geometric entities at asserted c
onnectivities');
#10227=UNCERTAINTY_MEASURE_WITH_UNIT(LENGTH_MEASURE(0.001),#10266,
'DISTANCE_ACCURACY_VALUE',
'Maximum model space distance between geometric entities at asserted c
onnectivities');
#10238=(
GEOMETRIC_REPRESENTATION_CONTEXT(3)
GLOBAL_UNCERTAINTY_ASSIGNED_CONTEXT((#10200))
GLOBAL_UNIT_ASSIGNED_CONTEXT((#10266,#10268,#10269))
REPRESENTATION_CONTEXT('','3D')
);
#10265=(
GEOMETRIC_REPRESENTATION_CONTEXT(3)
GLOBAL_UNCERTAINTY_ASSIGNED_CONTEXT((#10227))
GLOBAL_UNIT_ASSIGNED_CONTEXT((#10266,#10268,#10269))
REPRESENTATION_CONTEXT('','3D')
);
#10266=(
LENGTH_UNIT()
NAMED_UNIT(*)
SI_UNIT(.CENTI.,.METRE.)
);
#10268=(
NAMED_UNIT(*)
PLANE_ANGLE_UNIT()
SI_UNIT($,.RADIAN.)
);
#10269=(
NAMED_UNIT(*)
SI_UNIT($,.STERADIAN.)
SOLID_ANGLE_UNIT()
);
#10280=SHAPE_DEFINITION_REPRESENTATION(#10317,#10414);
#10317=PRODUCT_DEFINITION_SHAPE('',$,#10452);
#10414=SHAPE_REPRESENTATION('',(#5597),#10238);
#10441=PRODUCT_DEFINITION_CONTEXT('part definition',#10554,'design');
#10452=PRODUCT_DEFINITION('Cylinder bottom cap','Cylinder bottom cap',#10489,
#10441);
#10489=PRODUCT_DEFINITION_FORMATION('',$,#10566);
#10554=APPLICATION_CONTEXT(
'Core Data for Automotive Mechanical Design Process');
#10555=PRODUCT_CONTEXT('part definition',#10554,'mechanical');
#10566=PRODUCT('Cylinder bottom cap','Cylinder bottom cap',
'Cylinder bottom cap',(#10555));
#10642=COLOUR_RGB('Sky Blue',0.24,0.69,0.87);
#10643=FILL_AREA_STYLE_COLOUR('',#10642);
#10644=FILL_AREA_STYLE('',(#10643));
#10645=SURFACE_STYLE_FILL_AREA(#10644);
#10646=SURFACE_SIDE_STYLE('',(#10645));
#10647=SURFACE_STYLE_USAGE(.BOTH.,#10646);
#10648=PRESENTATION_STYLE_ASSIGNMENT((#10647));
ENDSEC;
END-ISO-10303-21;
